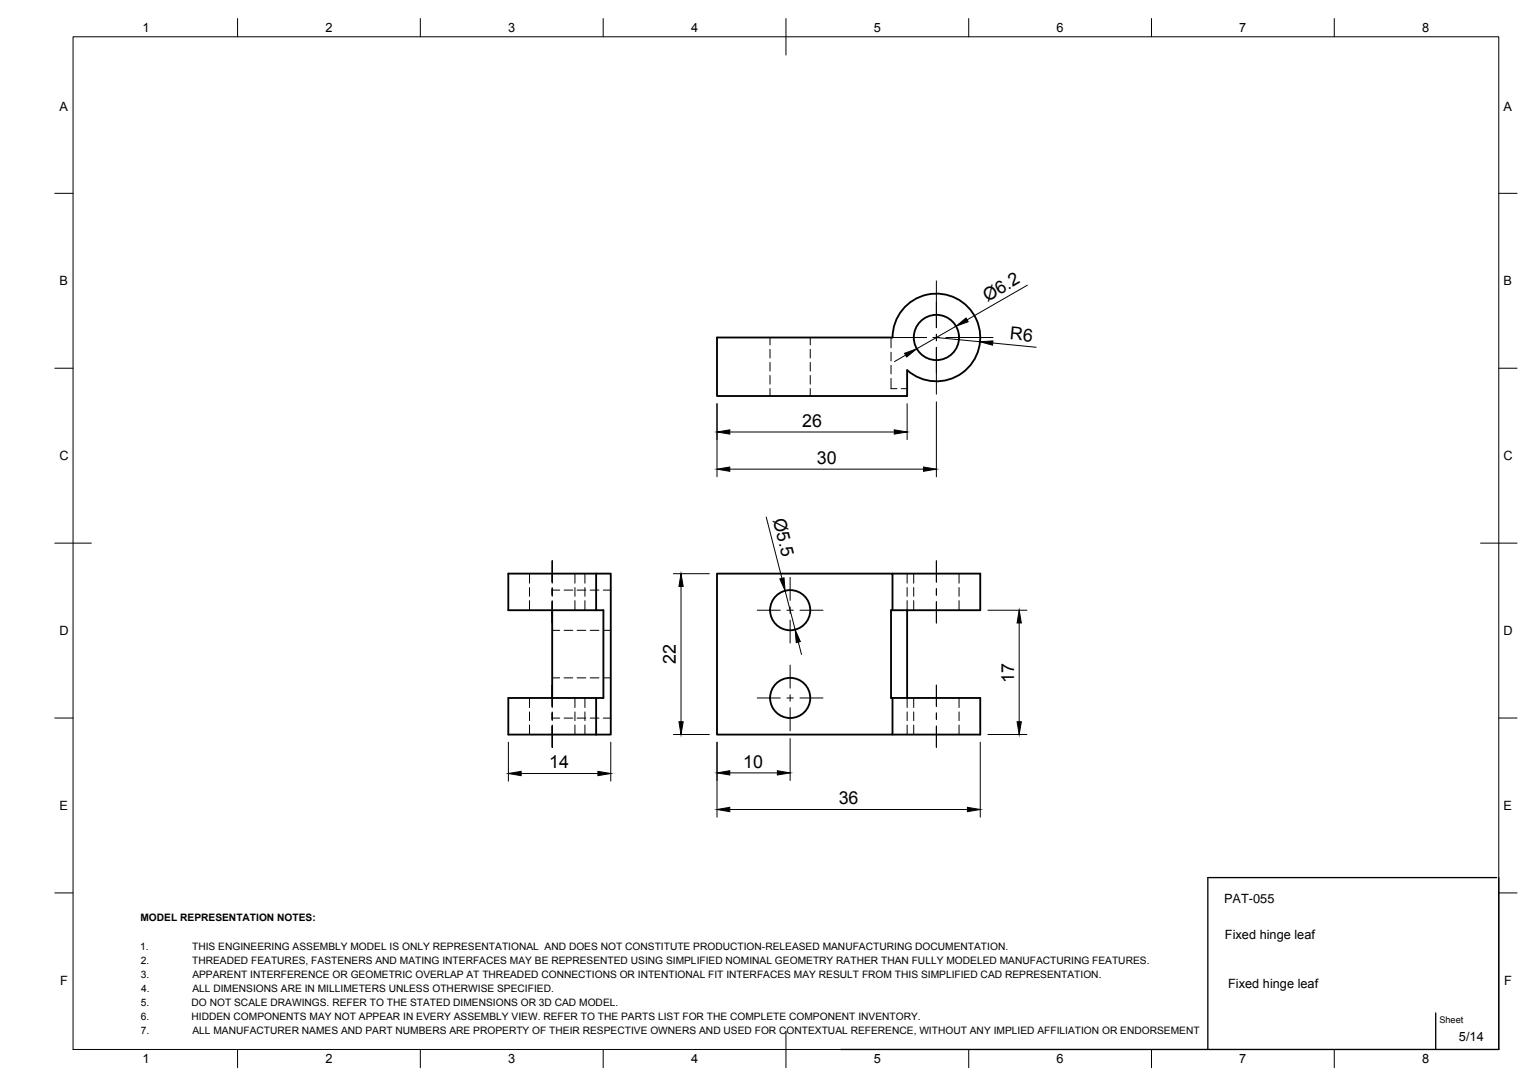
ISO-10303-21;
HEADER;
/* Generated by software containing ST-Developer
 * from STEP Tools, Inc. (www.steptools.com) 
 */

FILE_DESCRIPTION(
/* description */ ('Hinged panel with latch'),
/* implementation_level */ '2;1');

FILE_NAME(
/* name */ 'Fixed hinge leaf.step',
/* time_stamp */ '2026-10-27T20:36:01-07:00',
/* author */ (''),
/* organization */ (''),
/* preprocessor_version */ 'ST-DEVELOPER v20.2',
/* originating_system */ 'Autodesk Translation Framework v15.17.0.0',
/* authorisation */ '');

FILE_SCHEMA (('AUTOMOTIVE_DESIGN { 1 0 10303 214 3 1 1 }'));
ENDSEC;

DATA;
#10=MECHANICAL_DESIGN_GEOMETRIC_PRESENTATION_REPRESENTATION('',(#298),#6743);
#266=SHAPE_REPRESENTATION_RELATIONSHIP('SRR','None',#6841,#282);
#282=ADVANCED_BREP_SHAPE_REPRESENTATION('',(#314),#6727);
#298=STYLED_ITEM('',(#6989),#314);
#314=MANIFOLD_SOLID_BREP('Body1',#3800);
#331=FACE_BOUND('',#797,.T.);
#332=FACE_BOUND('',#798,.T.);
#333=FACE_BOUND('',#801,.T.);
#334=FACE_BOUND('',#804,.T.);
#335=FACE_BOUND('',#807,.T.);
#336=FACE_BOUND('',#809,.T.);
#337=FACE_BOUND('',#810,.T.);
#338=FACE_BOUND('',#813,.T.);
#424=PLANE('',#4072);
#425=PLANE('',#4073);
#426=PLANE('',#4074);
#427=PLANE('',#4078);
#428=PLANE('',#4079);
#429=PLANE('',#4080);
#430=PLANE('',#4084);
#431=PLANE('',#4085);
#432=PLANE('',#4086);
#433=PLANE('',#4087);
#578=FACE_OUTER_BOUND('',#790,.T.);
#579=FACE_OUTER_BOUND('',#791,.T.);
#580=FACE_OUTER_BOUND('',#792,.T.);
#581=FACE_OUTER_BOUND('',#793,.T.);
#582=FACE_OUTER_BOUND('',#794,.T.);
#583=FACE_OUTER_BOUND('',#795,.T.);
#584=FACE_OUTER_BOUND('',#796,.T.);
#585=FACE_OUTER_BOUND('',#799,.T.);
#586=FACE_OUTER_BOUND('',#800,.T.);
#587=FACE_OUTER_BOUND('',#802,.T.);
#588=FACE_OUTER_BOUND('',#803,.T.);
#589=FACE_OUTER_BOUND('',#805,.T.);
#590=FACE_OUTER_BOUND('',#806,.T.);
#591=FACE_OUTER_BOUND('',#808,.T.);
#592=FACE_OUTER_BOUND('',#811,.T.);
#593=FACE_OUTER_BOUND('',#812,.T.);
#790=EDGE_LOOP('',(#2896,#2897,#2898,#2899));
#791=EDGE_LOOP('',(#2900,#2901,#2902,#2903));
#792=EDGE_LOOP('',(#2904,#2905,#2906,#2907));
#793=EDGE_LOOP('',(#2908,#2909,#2910,#2911));
#794=EDGE_LOOP('',(#2912,#2913,#2914,#2915));
#795=EDGE_LOOP('',(#2916,#2917,#2918,#2919));
#796=EDGE_LOOP('',(#2920,#2921,#2922,#2923,#2924,#2925,#2926,#2927));
#797=EDGE_LOOP('',(#2928));
#798=EDGE_LOOP('',(#2929));
#799=EDGE_LOOP('',(#2930,#2931,#2932,#2933));
#800=EDGE_LOOP('',(#2934,#2935,#2936,#2937,#2938));
#801=EDGE_LOOP('',(#2939));
#802=EDGE_LOOP('',(#2940,#2941,#2942,#2943,#2944,#2945,#2946,#2947));
#803=EDGE_LOOP('',(#2948,#2949,#2950,#2951,#2952));
#804=EDGE_LOOP('',(#2953));
#805=EDGE_LOOP('',(#2954,#2955,#2956,#2957));
#806=EDGE_LOOP('',(#2958,#2959,#2960,#2961,#2962));
#807=EDGE_LOOP('',(#2963));
#808=EDGE_LOOP('',(#2964,#2965,#2966,#2967));
#809=EDGE_LOOP('',(#2968));
#810=EDGE_LOOP('',(#2969));
#811=EDGE_LOOP('',(#2970,#2971,#2972,#2973));
#812=EDGE_LOOP('',(#2974,#2975,#2976,#2977,#2978));
#813=EDGE_LOOP('',(#2979));
#1129=LINE('',#5781,#1487);
#1130=LINE('',#5787,#1488);
#1131=LINE('',#5793,#1489);
#1132=LINE('',#5799,#1490);
#1133=LINE('',#5804,#1491);
#1134=LINE('',#5806,#1492);
#1135=LINE('',#5808,#1493);
#1136=LINE('',#5809,#1494);
#1137=LINE('',#5813,#1495);
#1138=LINE('',#5814,#1496);
#1139=LINE('',#5815,#1497);
#1140=LINE('',#5818,#1498);
#1141=LINE('',#5820,#1499);
#1142=LINE('',#5822,#1500);
#1143=LINE('',#5824,#1501);
#1144=LINE('',#5826,#1502);
#1145=LINE('',#5828,#1503);
#1146=LINE('',#5829,#1504);
#1147=LINE('',#5833,#1505);
#1148=LINE('',#5837,#1506);
#1149=LINE('',#5840,#1507);
#1150=LINE('',#5842,#1508);
#1151=LINE('',#5844,#1509);
#1152=LINE('',#5846,#1510);
#1153=LINE('',#5847,#1511);
#1154=LINE('',#5854,#1512);
#1155=LINE('',#5855,#1513);
#1156=LINE('',#5858,#1514);
#1157=LINE('',#5859,#1515);
#1158=LINE('',#5861,#1516);
#1487=VECTOR('',#4647,0.275);
#1488=VECTOR('',#4654,0.275);
#1489=VECTOR('',#4661,0.31);
#1490=VECTOR('',#4668,0.31);
#1491=VECTOR('',#4673,1.);
#1492=VECTOR('',#4674,1.);
#1493=VECTOR('',#4675,1.);
#1494=VECTOR('',#4676,1.);
#1495=VECTOR('',#4679,1.);
#1496=VECTOR('',#4680,1.);
#1497=VECTOR('',#4681,1.);
#1498=VECTOR('',#4684,1.);
#1499=VECTOR('',#4685,1.);
#1500=VECTOR('',#4686,1.);
#1501=VECTOR('',#4687,1.);
#1502=VECTOR('',#4688,1.);
#1503=VECTOR('',#4689,1.);
#1504=VECTOR('',#4690,1.);
#1505=VECTOR('',#4693,1.);
#1506=VECTOR('',#4700,1.);
#1507=VECTOR('',#4703,1.);
#1508=VECTOR('',#4704,1.);
#1509=VECTOR('',#4705,1.);
#1510=VECTOR('',#4706,1.);
#1511=VECTOR('',#4707,1.);
#1512=VECTOR('',#4718,1.);
#1513=VECTOR('',#4719,1.);
#1514=VECTOR('',#4722,1.);
#1515=VECTOR('',#4723,1.);
#1516=VECTOR('',#4726,1.);
#1704=CIRCLE('',#4061,0.275);
#1705=CIRCLE('',#4062,0.275);
#1706=CIRCLE('',#4064,0.275);
#1707=CIRCLE('',#4065,0.275);
#1708=CIRCLE('',#4067,0.31);
#1709=CIRCLE('',#4068,0.31);
#1710=CIRCLE('',#4070,0.31);
#1711=CIRCLE('',#4071,0.31);
#1712=CIRCLE('',#4076,0.6);
#1713=CIRCLE('',#4077,0.6);
#1714=CIRCLE('',#4081,0.6);
#1715=CIRCLE('',#4083,0.6);
#1893=VERTEX_POINT('',#5778);
#1894=VERTEX_POINT('',#5780);
#1895=VERTEX_POINT('',#5784);
#1896=VERTEX_POINT('',#5786);
#1897=VERTEX_POINT('',#5790);
#1898=VERTEX_POINT('',#5792);
#1899=VERTEX_POINT('',#5796);
#1900=VERTEX_POINT('',#5798);
#1901=VERTEX_POINT('',#5802);
#1902=VERTEX_POINT('',#5803);
#1903=VERTEX_POINT('',#5805);
#1904=VERTEX_POINT('',#5807);
#1905=VERTEX_POINT('',#5811);
#1906=VERTEX_POINT('',#5812);
#1907=VERTEX_POINT('',#5817);
#1908=VERTEX_POINT('',#5819);
#1909=VERTEX_POINT('',#5821);
#1910=VERTEX_POINT('',#5823);
#1911=VERTEX_POINT('',#5825);
#1912=VERTEX_POINT('',#5827);
#1913=VERTEX_POINT('',#5831);
#1914=VERTEX_POINT('',#5832);
#1915=VERTEX_POINT('',#5839);
#1916=VERTEX_POINT('',#5841);
#1917=VERTEX_POINT('',#5843);
#1918=VERTEX_POINT('',#5845);
#1919=VERTEX_POINT('',#5853);
#1920=VERTEX_POINT('',#5857);
#2260=EDGE_CURVE('',#1893,#1893,#1704,.T.);
#2261=EDGE_CURVE('',#1893,#1894,#1129,.T.);
#2262=EDGE_CURVE('',#1894,#1894,#1705,.T.);
#2263=EDGE_CURVE('',#1895,#1895,#1706,.T.);
#2264=EDGE_CURVE('',#1895,#1896,#1130,.T.);
#2265=EDGE_CURVE('',#1896,#1896,#1707,.T.);
#2266=EDGE_CURVE('',#1897,#1897,#1708,.T.);
#2267=EDGE_CURVE('',#1897,#1898,#1131,.T.);
#2268=EDGE_CURVE('',#1898,#1898,#1709,.T.);
#2269=EDGE_CURVE('',#1899,#1899,#1710,.T.);
#2270=EDGE_CURVE('',#1899,#1900,#1132,.T.);
#2271=EDGE_CURVE('',#1900,#1900,#1711,.T.);
#2272=EDGE_CURVE('',#1901,#1902,#1133,.T.);
#2273=EDGE_CURVE('',#1903,#1901,#1134,.T.);
#2274=EDGE_CURVE('',#1903,#1904,#1135,.T.);
#2275=EDGE_CURVE('',#1904,#1902,#1136,.T.);
#2276=EDGE_CURVE('',#1905,#1906,#1137,.T.);
#2277=EDGE_CURVE('',#1905,#1904,#1138,.T.);
#2278=EDGE_CURVE('',#1906,#1903,#1139,.T.);
#2279=EDGE_CURVE('',#1907,#1901,#1140,.T.);
#2280=EDGE_CURVE('',#1902,#1908,#1141,.T.);
#2281=EDGE_CURVE('',#1908,#1909,#1142,.T.);
#2282=EDGE_CURVE('',#1910,#1909,#1143,.T.);
#2283=EDGE_CURVE('',#1911,#1910,#1144,.T.);
#2284=EDGE_CURVE('',#1911,#1912,#1145,.T.);
#2285=EDGE_CURVE('',#1912,#1907,#1146,.T.);
#2286=EDGE_CURVE('',#1913,#1914,#1147,.T.);
#2287=EDGE_CURVE('',#1909,#1913,#1712,.T.);
#2288=EDGE_CURVE('',#1908,#1914,#1713,.T.);
#2289=EDGE_CURVE('',#1914,#1905,#1148,.T.);
#2290=EDGE_CURVE('',#1906,#1915,#1149,.T.);
#2291=EDGE_CURVE('',#1915,#1916,#1150,.T.);
#2292=EDGE_CURVE('',#1916,#1917,#1151,.T.);
#2293=EDGE_CURVE('',#1917,#1918,#1152,.T.);
#2294=EDGE_CURVE('',#1913,#1918,#1153,.T.);
#2295=EDGE_CURVE('',#1907,#1915,#1714,.T.);
#2296=EDGE_CURVE('',#1912,#1916,#1715,.T.);
#2297=EDGE_CURVE('',#1919,#1911,#1154,.T.);
#2298=EDGE_CURVE('',#1917,#1919,#1155,.T.);
#2299=EDGE_CURVE('',#1919,#1920,#1156,.T.);
#2300=EDGE_CURVE('',#1918,#1920,#1157,.T.);
#2301=EDGE_CURVE('',#1920,#1910,#1158,.T.);
#2896=ORIENTED_EDGE('',*,*,#2260,.F.);
#2897=ORIENTED_EDGE('',*,*,#2261,.T.);
#2898=ORIENTED_EDGE('',*,*,#2262,.F.);
#2899=ORIENTED_EDGE('',*,*,#2261,.F.);
#2900=ORIENTED_EDGE('',*,*,#2263,.F.);
#2901=ORIENTED_EDGE('',*,*,#2264,.T.);
#2902=ORIENTED_EDGE('',*,*,#2265,.F.);
#2903=ORIENTED_EDGE('',*,*,#2264,.F.);
#2904=ORIENTED_EDGE('',*,*,#2266,.F.);
#2905=ORIENTED_EDGE('',*,*,#2267,.T.);
#2906=ORIENTED_EDGE('',*,*,#2268,.F.);
#2907=ORIENTED_EDGE('',*,*,#2267,.F.);
#2908=ORIENTED_EDGE('',*,*,#2269,.F.);
#2909=ORIENTED_EDGE('',*,*,#2270,.T.);
#2910=ORIENTED_EDGE('',*,*,#2271,.F.);
#2911=ORIENTED_EDGE('',*,*,#2270,.F.);
#2912=ORIENTED_EDGE('',*,*,#2272,.F.);
#2913=ORIENTED_EDGE('',*,*,#2273,.F.);
#2914=ORIENTED_EDGE('',*,*,#2274,.T.);
#2915=ORIENTED_EDGE('',*,*,#2275,.T.);
#2916=ORIENTED_EDGE('',*,*,#2276,.F.);
#2917=ORIENTED_EDGE('',*,*,#2277,.T.);
#2918=ORIENTED_EDGE('',*,*,#2274,.F.);
#2919=ORIENTED_EDGE('',*,*,#2278,.F.);
#2920=ORIENTED_EDGE('',*,*,#2279,.T.);
#2921=ORIENTED_EDGE('',*,*,#2272,.T.);
#2922=ORIENTED_EDGE('',*,*,#2280,.T.);
#2923=ORIENTED_EDGE('',*,*,#2281,.T.);
#2924=ORIENTED_EDGE('',*,*,#2282,.F.);
#2925=ORIENTED_EDGE('',*,*,#2283,.F.);
#2926=ORIENTED_EDGE('',*,*,#2284,.T.);
#2927=ORIENTED_EDGE('',*,*,#2285,.T.);
#2928=ORIENTED_EDGE('',*,*,#2260,.T.);
#2929=ORIENTED_EDGE('',*,*,#2263,.T.);
#2930=ORIENTED_EDGE('',*,*,#2286,.F.);
#2931=ORIENTED_EDGE('',*,*,#2287,.F.);
#2932=ORIENTED_EDGE('',*,*,#2281,.F.);
#2933=ORIENTED_EDGE('',*,*,#2288,.T.);
#2934=ORIENTED_EDGE('',*,*,#2288,.F.);
#2935=ORIENTED_EDGE('',*,*,#2280,.F.);
#2936=ORIENTED_EDGE('',*,*,#2275,.F.);
#2937=ORIENTED_EDGE('',*,*,#2277,.F.);
#2938=ORIENTED_EDGE('',*,*,#2289,.F.);
#2939=ORIENTED_EDGE('',*,*,#2269,.T.);
#2940=ORIENTED_EDGE('',*,*,#2290,.T.);
#2941=ORIENTED_EDGE('',*,*,#2291,.T.);
#2942=ORIENTED_EDGE('',*,*,#2292,.T.);
#2943=ORIENTED_EDGE('',*,*,#2293,.T.);
#2944=ORIENTED_EDGE('',*,*,#2294,.F.);
#2945=ORIENTED_EDGE('',*,*,#2286,.T.);
#2946=ORIENTED_EDGE('',*,*,#2289,.T.);
#2947=ORIENTED_EDGE('',*,*,#2276,.T.);
#2948=ORIENTED_EDGE('',*,*,#2290,.F.);
#2949=ORIENTED_EDGE('',*,*,#2278,.T.);
#2950=ORIENTED_EDGE('',*,*,#2273,.T.);
#2951=ORIENTED_EDGE('',*,*,#2279,.F.);
#2952=ORIENTED_EDGE('',*,*,#2295,.T.);
#2953=ORIENTED_EDGE('',*,*,#2268,.T.);
#2954=ORIENTED_EDGE('',*,*,#2291,.F.);
#2955=ORIENTED_EDGE('',*,*,#2295,.F.);
#2956=ORIENTED_EDGE('',*,*,#2285,.F.);
#2957=ORIENTED_EDGE('',*,*,#2296,.T.);
#2958=ORIENTED_EDGE('',*,*,#2284,.F.);
#2959=ORIENTED_EDGE('',*,*,#2297,.F.);
#2960=ORIENTED_EDGE('',*,*,#2298,.F.);
#2961=ORIENTED_EDGE('',*,*,#2292,.F.);
#2962=ORIENTED_EDGE('',*,*,#2296,.F.);
#2963=ORIENTED_EDGE('',*,*,#2266,.T.);
#2964=ORIENTED_EDGE('',*,*,#2298,.T.);
#2965=ORIENTED_EDGE('',*,*,#2299,.T.);
#2966=ORIENTED_EDGE('',*,*,#2300,.F.);
#2967=ORIENTED_EDGE('',*,*,#2293,.F.);
#2968=ORIENTED_EDGE('',*,*,#2262,.T.);
#2969=ORIENTED_EDGE('',*,*,#2265,.T.);
#2970=ORIENTED_EDGE('',*,*,#2297,.T.);
#2971=ORIENTED_EDGE('',*,*,#2283,.T.);
#2972=ORIENTED_EDGE('',*,*,#2301,.F.);
#2973=ORIENTED_EDGE('',*,*,#2299,.F.);
#2974=ORIENTED_EDGE('',*,*,#2294,.T.);
#2975=ORIENTED_EDGE('',*,*,#2300,.T.);
#2976=ORIENTED_EDGE('',*,*,#2301,.T.);
#2977=ORIENTED_EDGE('',*,*,#2282,.T.);
#2978=ORIENTED_EDGE('',*,*,#2287,.T.);
#2979=ORIENTED_EDGE('',*,*,#2271,.T.);
#3559=CYLINDRICAL_SURFACE('',#4060,0.275);
#3560=CYLINDRICAL_SURFACE('',#4063,0.275);
#3561=CYLINDRICAL_SURFACE('',#4066,0.31);
#3562=CYLINDRICAL_SURFACE('',#4069,0.31);
#3563=CYLINDRICAL_SURFACE('',#4075,0.6);
#3564=CYLINDRICAL_SURFACE('',#4082,0.6);
#3647=ADVANCED_FACE('',(#578),#3559,.F.);
#3648=ADVANCED_FACE('',(#579),#3560,.F.);
#3649=ADVANCED_FACE('',(#580),#3561,.F.);
#3650=ADVANCED_FACE('',(#581),#3562,.F.);
#3651=ADVANCED_FACE('',(#582),#424,.F.);
#3652=ADVANCED_FACE('',(#583),#425,.F.);
#3653=ADVANCED_FACE('',(#584,#331,#332),#426,.T.);
#3654=ADVANCED_FACE('',(#585),#3563,.T.);
#3655=ADVANCED_FACE('',(#586,#333),#427,.F.);
#3656=ADVANCED_FACE('',(#587),#428,.T.);
#3657=ADVANCED_FACE('',(#588,#334),#429,.T.);
#3658=ADVANCED_FACE('',(#589),#3564,.T.);
#3659=ADVANCED_FACE('',(#590,#335),#430,.F.);
#3660=ADVANCED_FACE('',(#591,#336,#337),#431,.T.);
#3661=ADVANCED_FACE('',(#592),#432,.T.);
#3662=ADVANCED_FACE('',(#593,#338),#433,.T.);
#3800=CLOSED_SHELL('',(#3647,#3648,#3649,#3650,#3651,#3652,#3653,#3654,
#3655,#3656,#3657,#3658,#3659,#3660,#3661,#3662));
#4059=AXIS2_PLACEMENT_3D('',#5776,#4641,#4642);
#4060=AXIS2_PLACEMENT_3D('',#5777,#4643,#4644);
#4061=AXIS2_PLACEMENT_3D('',#5779,#4645,#4646);
#4062=AXIS2_PLACEMENT_3D('',#5782,#4648,#4649);
#4063=AXIS2_PLACEMENT_3D('',#5783,#4650,#4651);
#4064=AXIS2_PLACEMENT_3D('',#5785,#4652,#4653);
#4065=AXIS2_PLACEMENT_3D('',#5788,#4655,#4656);
#4066=AXIS2_PLACEMENT_3D('',#5789,#4657,#4658);
#4067=AXIS2_PLACEMENT_3D('',#5791,#4659,#4660);
#4068=AXIS2_PLACEMENT_3D('',#5794,#4662,#4663);
#4069=AXIS2_PLACEMENT_3D('',#5795,#4664,#4665);
#4070=AXIS2_PLACEMENT_3D('',#5797,#4666,#4667);
#4071=AXIS2_PLACEMENT_3D('',#5800,#4669,#4670);
#4072=AXIS2_PLACEMENT_3D('',#5801,#4671,#4672);
#4073=AXIS2_PLACEMENT_3D('',#5810,#4677,#4678);
#4074=AXIS2_PLACEMENT_3D('',#5816,#4682,#4683);
#4075=AXIS2_PLACEMENT_3D('',#5830,#4691,#4692);
#4076=AXIS2_PLACEMENT_3D('',#5834,#4694,#4695);
#4077=AXIS2_PLACEMENT_3D('',#5835,#4696,#4697);
#4078=AXIS2_PLACEMENT_3D('',#5836,#4698,#4699);
#4079=AXIS2_PLACEMENT_3D('',#5838,#4701,#4702);
#4080=AXIS2_PLACEMENT_3D('',#5848,#4708,#4709);
#4081=AXIS2_PLACEMENT_3D('',#5849,#4710,#4711);
#4082=AXIS2_PLACEMENT_3D('',#5850,#4712,#4713);
#4083=AXIS2_PLACEMENT_3D('',#5851,#4714,#4715);
#4084=AXIS2_PLACEMENT_3D('',#5852,#4716,#4717);
#4085=AXIS2_PLACEMENT_3D('',#5856,#4720,#4721);
#4086=AXIS2_PLACEMENT_3D('',#5860,#4724,#4725);
#4087=AXIS2_PLACEMENT_3D('',#5862,#4727,#4728);
#4641=DIRECTION('axis',(0.,0.,1.));
#4642=DIRECTION('refdir',(1.,0.,0.));
#4643=DIRECTION('center_axis',(0.,1.,0.));
#4644=DIRECTION('ref_axis',(1.,0.,0.));
#4645=DIRECTION('center_axis',(0.,1.,0.));
#4646=DIRECTION('ref_axis',(1.,0.,0.));
#4647=DIRECTION('',(0.,1.,0.));
#4648=DIRECTION('center_axis',(0.,-1.,0.));
#4649=DIRECTION('ref_axis',(1.,0.,0.));
#4650=DIRECTION('center_axis',(0.,1.,0.));
#4651=DIRECTION('ref_axis',(1.,0.,0.));
#4652=DIRECTION('center_axis',(0.,1.,0.));
#4653=DIRECTION('ref_axis',(1.,0.,0.));
#4654=DIRECTION('',(0.,1.,0.));
#4655=DIRECTION('center_axis',(0.,-1.,0.));
#4656=DIRECTION('ref_axis',(1.,0.,0.));
#4657=DIRECTION('center_axis',(0.,0.,1.));
#4658=DIRECTION('ref_axis',(1.,0.,0.));
#4659=DIRECTION('center_axis',(0.,0.,1.));
#4660=DIRECTION('ref_axis',(1.,0.,0.));
#4661=DIRECTION('',(0.,0.,1.));
#4662=DIRECTION('center_axis',(0.,0.,-1.));
#4663=DIRECTION('ref_axis',(1.,0.,0.));
#4664=DIRECTION('center_axis',(0.,0.,1.));
#4665=DIRECTION('ref_axis',(1.,0.,0.));
#4666=DIRECTION('center_axis',(0.,0.,1.));
#4667=DIRECTION('ref_axis',(1.,0.,0.));
#4668=DIRECTION('',(0.,0.,1.));
#4669=DIRECTION('center_axis',(0.,0.,-1.));
#4670=DIRECTION('ref_axis',(1.,0.,0.));
#4671=DIRECTION('center_axis',(-1.,0.,0.));
#4672=DIRECTION('ref_axis',(0.,-1.,0.));
#4673=DIRECTION('',(0.,0.,1.));
#4674=DIRECTION('',(0.,-1.,0.));
#4675=DIRECTION('',(0.,0.,1.));
#4676=DIRECTION('',(0.,-1.,0.));
#4677=DIRECTION('center_axis',(0.,1.,0.));
#4678=DIRECTION('ref_axis',(-1.,0.,0.));
#4679=DIRECTION('',(0.,0.,-1.));
#4680=DIRECTION('',(-1.,0.,0.));
#4681=DIRECTION('',(-1.,0.,0.));
#4682=DIRECTION('center_axis',(0.,-1.,0.));
#4683=DIRECTION('ref_axis',(1.,0.,0.));
#4684=DIRECTION('',(-1.,0.,0.));
#4685=DIRECTION('',(1.,0.,0.));
#4686=DIRECTION('',(0.,0.,1.));
#4687=DIRECTION('',(1.,0.,0.));
#4688=DIRECTION('',(0.,0.,1.));
#4689=DIRECTION('',(1.,0.,0.));
#4690=DIRECTION('',(0.,0.,1.));
#4691=DIRECTION('center_axis',(0.,0.,1.));
#4692=DIRECTION('ref_axis',(1.,0.,0.));
#4693=DIRECTION('',(0.,0.,-1.));
#4694=DIRECTION('center_axis',(0.,0.,1.));
#4695=DIRECTION('ref_axis',(1.,0.,0.));
#4696=DIRECTION('center_axis',(0.,0.,1.));
#4697=DIRECTION('ref_axis',(1.,0.,0.));
#4698=DIRECTION('center_axis',(0.,0.,1.));
#4699=DIRECTION('ref_axis',(1.,0.,0.));
#4700=DIRECTION('',(0.,1.,0.));
#4701=DIRECTION('center_axis',(1.,0.,0.));
#4702=DIRECTION('ref_axis',(0.,1.,0.));
#4703=DIRECTION('',(0.,-1.,0.));
#4704=DIRECTION('',(0.,0.,-1.));
#4705=DIRECTION('',(0.,1.,0.));
#4706=DIRECTION('',(0.,0.,1.));
#4707=DIRECTION('',(0.,1.,0.));
#4708=DIRECTION('center_axis',(0.,0.,1.));
#4709=DIRECTION('ref_axis',(1.,0.,0.));
#4710=DIRECTION('center_axis',(0.,0.,1.));
#4711=DIRECTION('ref_axis',(1.,0.,0.));
#4712=DIRECTION('center_axis',(0.,0.,1.));
#4713=DIRECTION('ref_axis',(1.,0.,0.));
#4714=DIRECTION('center_axis',(0.,0.,1.));
#4715=DIRECTION('ref_axis',(1.,0.,0.));
#4716=DIRECTION('center_axis',(0.,0.,1.));
#4717=DIRECTION('ref_axis',(1.,0.,0.));
#4718=DIRECTION('',(0.,-1.,0.));
#4719=DIRECTION('',(-1.,0.,0.));
#4720=DIRECTION('center_axis',(0.,1.,0.));
#4721=DIRECTION('ref_axis',(-1.,0.,0.));
#4722=DIRECTION('',(0.,0.,1.));
#4723=DIRECTION('',(-1.,0.,0.));
#4724=DIRECTION('center_axis',(-1.,0.,0.));
#4725=DIRECTION('ref_axis',(0.,-1.,0.));
#4726=DIRECTION('',(0.,-1.,0.));
#4727=DIRECTION('center_axis',(0.,0.,1.));
#4728=DIRECTION('ref_axis',(1.,0.,0.));
#5776=CARTESIAN_POINT('',(0.,0.,0.));
#5777=CARTESIAN_POINT('Origin',(0.,-2.1,6.));
#5778=CARTESIAN_POINT('',(-0.275,-1.8,6.));
#5779=CARTESIAN_POINT('Origin',(0.,-1.8,6.));
#5780=CARTESIAN_POINT('',(-0.275,-1.,6.));
#5781=CARTESIAN_POINT('',(-0.275,-2.1,6.));
#5782=CARTESIAN_POINT('Origin',(0.,-1.,6.));
#5783=CARTESIAN_POINT('Origin',(0.,-2.1,7.2));
#5784=CARTESIAN_POINT('',(-0.275,-1.8,7.2));
#5785=CARTESIAN_POINT('Origin',(0.,-1.8,7.2));
#5786=CARTESIAN_POINT('',(-0.275,-1.,7.2));
#5787=CARTESIAN_POINT('',(-0.275,-2.1,7.2));
#5788=CARTESIAN_POINT('Origin',(0.,-1.,7.2));
#5789=CARTESIAN_POINT('Origin',(2.,-1.8,5.4));
#5790=CARTESIAN_POINT('',(1.69,-1.8,5.5));
#5791=CARTESIAN_POINT('Origin',(2.,-1.8,5.5));
#5792=CARTESIAN_POINT('',(1.69,-1.8,6.));
#5793=CARTESIAN_POINT('',(1.69,-1.8,5.4));
#5794=CARTESIAN_POINT('Origin',(2.,-1.8,6.));
#5795=CARTESIAN_POINT('Origin',(2.,-1.8,5.4));
#5796=CARTESIAN_POINT('',(1.69,-1.8,7.2));
#5797=CARTESIAN_POINT('Origin',(2.,-1.8,7.2));
#5798=CARTESIAN_POINT('',(1.69,-1.8,7.7));
#5799=CARTESIAN_POINT('',(1.69,-1.8,5.4));
#5800=CARTESIAN_POINT('Origin',(2.,-1.8,7.7));
#5801=CARTESIAN_POINT('Origin',(1.38,-1.1,6.));
#5802=CARTESIAN_POINT('',(1.38,-1.8,6.));
#5803=CARTESIAN_POINT('',(1.38,-1.8,7.2));
#5804=CARTESIAN_POINT('',(1.38,-1.8,5.75));
#5805=CARTESIAN_POINT('',(1.38,-1.1,6.));
#5806=CARTESIAN_POINT('',(1.38,-1.1,6.));
#5807=CARTESIAN_POINT('',(1.38,-1.1,7.2));
#5808=CARTESIAN_POINT('',(1.38,-1.1,6.));
#5809=CARTESIAN_POINT('',(1.38,-1.1,7.2));
#5810=CARTESIAN_POINT('Origin',(2.7,-1.1,6.));
#5811=CARTESIAN_POINT('',(1.6,-1.1,7.2));
#5812=CARTESIAN_POINT('',(1.6,-1.1,6.));
#5813=CARTESIAN_POINT('',(1.6,-1.1,5.75));
#5814=CARTESIAN_POINT('',(2.7,-1.1,7.2));
#5815=CARTESIAN_POINT('',(2.7,-1.1,6.));
#5816=CARTESIAN_POINT('Origin',(-1.,-1.8,5.5));
#5817=CARTESIAN_POINT('',(1.4,-1.8,6.));
#5818=CARTESIAN_POINT('',(0.52,-1.8,6.));
#5819=CARTESIAN_POINT('',(1.4,-1.8,7.2));
#5820=CARTESIAN_POINT('',(0.52,-1.8,7.2));
#5821=CARTESIAN_POINT('',(1.4,-1.8,7.7));
#5822=CARTESIAN_POINT('',(1.4,-1.8,7.2));
#5823=CARTESIAN_POINT('',(-1.,-1.8,7.7));
#5824=CARTESIAN_POINT('',(-1.,-1.8,7.7));
#5825=CARTESIAN_POINT('',(-1.,-1.8,5.5));
#5826=CARTESIAN_POINT('',(-1.,-1.8,5.5));
#5827=CARTESIAN_POINT('',(1.4,-1.8,5.5));
#5828=CARTESIAN_POINT('',(-1.,-1.8,5.5));
#5829=CARTESIAN_POINT('',(1.4,-1.8,5.5));
#5830=CARTESIAN_POINT('Origin',(2.,-1.8,7.2));
#5831=CARTESIAN_POINT('',(1.6,-1.35278640450004,7.7));
#5832=CARTESIAN_POINT('',(1.6,-1.35278640450004,7.2));
#5833=CARTESIAN_POINT('',(1.6,-1.35278640450004,7.2));
#5834=CARTESIAN_POINT('Origin',(2.,-1.8,7.7));
#5835=CARTESIAN_POINT('Origin',(2.,-1.8,7.2));
#5836=CARTESIAN_POINT('Origin',(2.,-1.8,7.2));
#5837=CARTESIAN_POINT('',(1.6,-1.8,7.2));
#5838=CARTESIAN_POINT('Origin',(1.6,-1.8,5.5));
#5839=CARTESIAN_POINT('',(1.6,-1.35278640450004,6.));
#5840=CARTESIAN_POINT('',(1.6,-1.8,6.));
#5841=CARTESIAN_POINT('',(1.6,-1.35278640450004,5.5));
#5842=CARTESIAN_POINT('',(1.6,-1.35278640450004,5.5));
#5843=CARTESIAN_POINT('',(1.6,-1.,5.5));
#5844=CARTESIAN_POINT('',(1.6,-1.8,5.5));
#5845=CARTESIAN_POINT('',(1.6,-1.,7.7));
#5846=CARTESIAN_POINT('',(1.6,-1.,5.5));
#5847=CARTESIAN_POINT('',(1.6,-1.8,7.7));
#5848=CARTESIAN_POINT('Origin',(2.,-1.8,6.));
#5849=CARTESIAN_POINT('Origin',(2.,-1.8,6.));
#5850=CARTESIAN_POINT('Origin',(2.,-1.8,5.5));
#5851=CARTESIAN_POINT('Origin',(2.,-1.8,5.5));
#5852=CARTESIAN_POINT('Origin',(0.3,-1.4,5.5));
#5853=CARTESIAN_POINT('',(-1.,-1.,5.5));
#5854=CARTESIAN_POINT('',(-1.,-1.,5.5));
#5855=CARTESIAN_POINT('',(1.6,-1.,5.5));
#5856=CARTESIAN_POINT('Origin',(1.6,-1.,5.5));
#5857=CARTESIAN_POINT('',(-1.,-1.,7.7));
#5858=CARTESIAN_POINT('',(-1.,-1.,5.5));
#5859=CARTESIAN_POINT('',(1.6,-1.,7.7));
#5860=CARTESIAN_POINT('Origin',(-1.,-1.,5.5));
#5861=CARTESIAN_POINT('',(-1.,-1.,7.7));
#5862=CARTESIAN_POINT('Origin',(0.3,-1.4,7.7));
#6706=UNCERTAINTY_MEASURE_WITH_UNIT(LENGTH_MEASURE(0.001),#6744,
'DISTANCE_ACCURACY_VALUE',
'Maximum model space distance between geometric entities at asserted c
onnectivities');
#6722=UNCERTAINTY_MEASURE_WITH_UNIT(LENGTH_MEASURE(0.001),#6744,
'DISTANCE_ACCURACY_VALUE',
'Maximum model space distance between geometric entities at asserted c
onnectivities');
#6727=(
GEOMETRIC_REPRESENTATION_CONTEXT(3)
GLOBAL_UNCERTAINTY_ASSIGNED_CONTEXT((#6706))
GLOBAL_UNIT_ASSIGNED_CONTEXT((#6744,#6746,#6747))
REPRESENTATION_CONTEXT('','3D')
);
#6743=(
GEOMETRIC_REPRESENTATION_CONTEXT(3)
GLOBAL_UNCERTAINTY_ASSIGNED_CONTEXT((#6722))
GLOBAL_UNIT_ASSIGNED_CONTEXT((#6744,#6746,#6747))
REPRESENTATION_CONTEXT('','3D')
);
#6744=(
LENGTH_UNIT()
NAMED_UNIT(*)
SI_UNIT(.CENTI.,.METRE.)
);
#6746=(
NAMED_UNIT(*)
PLANE_ANGLE_UNIT()
SI_UNIT($,.RADIAN.)
);
#6747=(
NAMED_UNIT(*)
SI_UNIT($,.STERADIAN.)
SOLID_ANGLE_UNIT()
);
#6752=SHAPE_DEFINITION_REPRESENTATION(#6772,#6841);
#6772=PRODUCT_DEFINITION_SHAPE('',$,#6862);
#6841=SHAPE_REPRESENTATION('',(#4059),#6727);
#6857=PRODUCT_DEFINITION_CONTEXT('part definition',#6919,'design');
#6862=PRODUCT_DEFINITION('Fixed hinge leaf','Fixed hinge leaf',#6882,#6857);
#6882=PRODUCT_DEFINITION_FORMATION('',$,#6925);
#6919=APPLICATION_CONTEXT(
'Core Data for Automotive Mechanical Design Process');
#6920=PRODUCT_CONTEXT('part definition',#6919,'mechanical');
#6925=PRODUCT('Fixed hinge leaf','Fixed hinge leaf','Fixed hinge leaf',
(#6920));
#6983=COLOUR_RGB('Light Blue',0.38,0.62,0.78);
#6984=FILL_AREA_STYLE_COLOUR('',#6983);
#6985=FILL_AREA_STYLE('',(#6984));
#6986=SURFACE_STYLE_FILL_AREA(#6985);
#6987=SURFACE_SIDE_STYLE('',(#6986));
#6988=SURFACE_STYLE_USAGE(.BOTH.,#6987);
#6989=PRESENTATION_STYLE_ASSIGNMENT((#6988));
ENDSEC;
END-ISO-10303-21;
